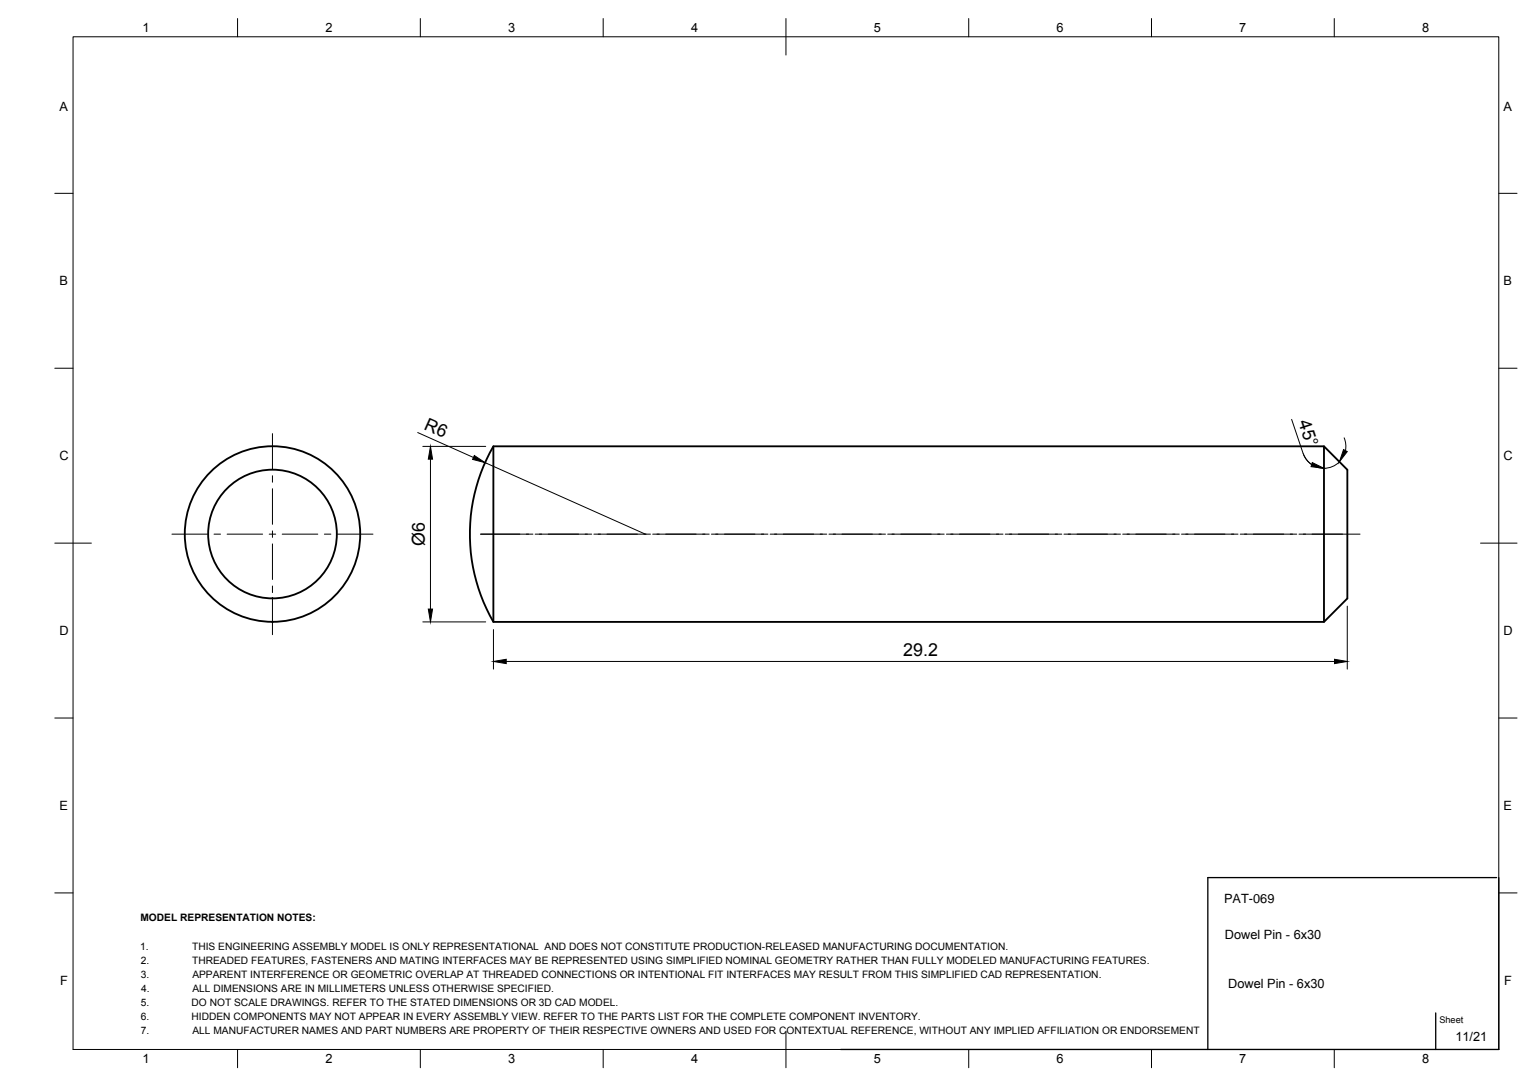
ISO-10303-21;
HEADER;
/* Generated by software containing ST-Developer
 * from STEP Tools, Inc. (www.steptools.com) 
 */

FILE_DESCRIPTION(
/* description */ ('Located fixture plate with toggle clamp'),
/* implementation_level */ '2;1');

FILE_NAME(
/* name */ 'Dowel Pin - 6x30.step',
/* time_stamp */ '2026-10-27T21:36:12-07:00',
/* author */ (''),
/* organization */ (''),
/* preprocessor_version */ 'ST-DEVELOPER v20.2',
/* originating_system */ 'Autodesk Translation Framework v15.17.0.0',
/* authorisation */ '');

FILE_SCHEMA (('AUTOMOTIVE_DESIGN { 1 0 10303 214 3 1 1 }'));
ENDSEC;

DATA;
#10=MECHANICAL_DESIGN_GEOMETRIC_PRESENTATION_REPRESENTATION('',(#330),#9285);
#202=SPHERICAL_SURFACE('',#5729,0.600000000000005);
#258=CONICAL_SURFACE('',#5733,0.26,0.785398163397448);
#282=SHAPE_REPRESENTATION_RELATIONSHIP('SRR','None',#9405,#306);
#306=ADVANCED_BREP_SHAPE_REPRESENTATION('',(#353),#9267);
#330=STYLED_ITEM('',(#9612),#353);
#353=MANIFOLD_SOLID_BREP('Body1',#5179);
#577=PLANE('',#5735);
#821=FACE_OUTER_BOUND('',#1202,.T.);
#822=FACE_OUTER_BOUND('',#1203,.T.);
#823=FACE_OUTER_BOUND('',#1204,.T.);
#824=FACE_OUTER_BOUND('',#1205,.T.);
#1202=EDGE_LOOP('',(#4188));
#1203=EDGE_LOOP('',(#4189,#4190,#4191,#4192));
#1204=EDGE_LOOP('',(#4193,#4194,#4195,#4196));
#1205=EDGE_LOOP('',(#4197));
#1491=CIRCLE('',#5730,0.3);
#1492=CIRCLE('',#5732,0.3);
#1493=CIRCLE('',#5734,0.22);
#1807=LINE('',#8361,#2217);
#1808=LINE('',#8365,#2218);
#2217=VECTOR('',#6799,0.3);
#2218=VECTOR('',#6804,0.26);
#2633=VERTEX_POINT('',#8356);
#2634=VERTEX_POINT('',#8359);
#2635=VERTEX_POINT('',#8363);
#3182=EDGE_CURVE('',#2633,#2633,#1491,.T.);
#3183=EDGE_CURVE('',#2634,#2634,#1492,.T.);
#3184=EDGE_CURVE('',#2634,#2633,#1807,.T.);
#3185=EDGE_CURVE('',#2635,#2635,#1493,.T.);
#3186=EDGE_CURVE('',#2635,#2634,#1808,.T.);
#4188=ORIENTED_EDGE('',*,*,#3182,.F.);
#4189=ORIENTED_EDGE('',*,*,#3183,.F.);
#4190=ORIENTED_EDGE('',*,*,#3184,.T.);
#4191=ORIENTED_EDGE('',*,*,#3182,.T.);
#4192=ORIENTED_EDGE('',*,*,#3184,.F.);
#4193=ORIENTED_EDGE('',*,*,#3185,.F.);
#4194=ORIENTED_EDGE('',*,*,#3186,.T.);
#4195=ORIENTED_EDGE('',*,*,#3183,.T.);
#4196=ORIENTED_EDGE('',*,*,#3186,.F.);
#4197=ORIENTED_EDGE('',*,*,#3185,.T.);
#4841=CYLINDRICAL_SURFACE('',#5731,0.3);
#5022=ADVANCED_FACE('',(#821),#202,.T.);
#5023=ADVANCED_FACE('',(#822),#4841,.T.);
#5024=ADVANCED_FACE('',(#823),#258,.T.);
#5025=ADVANCED_FACE('',(#824),#577,.T.);
#5179=CLOSED_SHELL('',(#5022,#5023,#5024,#5025));
#5728=AXIS2_PLACEMENT_3D('',#8354,#6789,#6790);
#5729=AXIS2_PLACEMENT_3D('',#8355,#6791,#6792);
#5730=AXIS2_PLACEMENT_3D('',#8357,#6793,#6794);
#5731=AXIS2_PLACEMENT_3D('',#8358,#6795,#6796);
#5732=AXIS2_PLACEMENT_3D('',#8360,#6797,#6798);
#5733=AXIS2_PLACEMENT_3D('',#8362,#6800,#6801);
#5734=AXIS2_PLACEMENT_3D('',#8364,#6802,#6803);
#5735=AXIS2_PLACEMENT_3D('',#8366,#6805,#6806);
#6789=DIRECTION('axis',(0.,0.,1.));
#6790=DIRECTION('refdir',(1.,0.,0.));
#6791=DIRECTION('center_axis',(6.12323399573677E-17,0.,1.));
#6792=DIRECTION('ref_axis',(1.,0.,0.));
#6793=DIRECTION('center_axis',(0.,-1.,0.));
#6794=DIRECTION('ref_axis',(1.,0.,0.));
#6795=DIRECTION('center_axis',(0.,-1.,0.));
#6796=DIRECTION('ref_axis',(1.,0.,0.));
#6797=DIRECTION('center_axis',(0.,-1.,0.));
#6798=DIRECTION('ref_axis',(1.,0.,0.));
#6799=DIRECTION('',(0.,1.,0.));
#6800=DIRECTION('center_axis',(0.,1.,0.));
#6801=DIRECTION('ref_axis',(1.,0.,0.));
#6802=DIRECTION('center_axis',(0.,-1.,0.));
#6803=DIRECTION('ref_axis',(1.,0.,0.));
#6804=DIRECTION('',(-0.707106781186547,0.707106781186548,-8.65956056235493E-17));
#6805=DIRECTION('center_axis',(0.,-1.,0.));
#6806=DIRECTION('ref_axis',(0.,0.,-1.));
#8354=CARTESIAN_POINT('',(0.,0.,0.));
#8355=CARTESIAN_POINT('Origin',(-8.04911692853238E-16,2.4,0.));
#8356=CARTESIAN_POINT('',(-0.3,2.91961524227066,-3.67394039744206E-17));
#8357=CARTESIAN_POINT('Origin',(0.,2.91961524227066,0.));
#8358=CARTESIAN_POINT('Origin',(0.,1.49980762113533,0.));
#8359=CARTESIAN_POINT('',(-0.3,0.0800000000000001,-3.67394039744206E-17));
#8360=CARTESIAN_POINT('Origin',(0.,0.08,0.));
#8361=CARTESIAN_POINT('',(-0.3,1.49980762113533,-3.67394039744206E-17));
#8362=CARTESIAN_POINT('Origin',(0.,0.04,0.));
#8363=CARTESIAN_POINT('',(-0.22,-6.93889390390723E-18,-2.69422295812418E-17));
#8364=CARTESIAN_POINT('Origin',(0.,0.,0.));
#8365=CARTESIAN_POINT('',(-0.26,0.04,-3.18408167778312E-17));
#8366=CARTESIAN_POINT('Origin',(0.,0.,0.));
#9237=UNCERTAINTY_MEASURE_WITH_UNIT(LENGTH_MEASURE(0.001),#9286,
'DISTANCE_ACCURACY_VALUE',
'Maximum model space distance between geometric entities at asserted c
onnectivities');
#9255=UNCERTAINTY_MEASURE_WITH_UNIT(LENGTH_MEASURE(0.001),#9286,
'DISTANCE_ACCURACY_VALUE',
'Maximum model space distance between geometric entities at asserted c
onnectivities');
#9267=(
GEOMETRIC_REPRESENTATION_CONTEXT(3)
GLOBAL_UNCERTAINTY_ASSIGNED_CONTEXT((#9237))
GLOBAL_UNIT_ASSIGNED_CONTEXT((#9286,#9288,#9289))
REPRESENTATION_CONTEXT('','3D')
);
#9285=(
GEOMETRIC_REPRESENTATION_CONTEXT(3)
GLOBAL_UNCERTAINTY_ASSIGNED_CONTEXT((#9255))
GLOBAL_UNIT_ASSIGNED_CONTEXT((#9286,#9288,#9289))
REPRESENTATION_CONTEXT('','3D')
);
#9286=(
LENGTH_UNIT()
NAMED_UNIT(*)
SI_UNIT(.CENTI.,.METRE.)
);
#9288=(
NAMED_UNIT(*)
PLANE_ANGLE_UNIT()
SI_UNIT($,.RADIAN.)
);
#9289=(
NAMED_UNIT(*)
SI_UNIT($,.STERADIAN.)
SOLID_ANGLE_UNIT()
);
#9301=SHAPE_DEFINITION_REPRESENTATION(#9330,#9405);
#9330=PRODUCT_DEFINITION_SHAPE('',$,#9435);
#9405=SHAPE_REPRESENTATION('',(#5728),#9267);
#9423=PRODUCT_DEFINITION_CONTEXT('part definition',#9512,'design');
#9435=PRODUCT_DEFINITION('Dowel Pin - 6x30','Dowel Pin - 6x30',#9464,#9423);
#9464=PRODUCT_DEFINITION_FORMATION('',$,#9525);
#9512=APPLICATION_CONTEXT(
'Core Data for Automotive Mechanical Design Process');
#9513=PRODUCT_CONTEXT('part definition',#9512,'mechanical');
#9525=PRODUCT('Dowel Pin - 6x30','Dowel Pin - 6x30','Dowel Pin - 6x30',
(#9513));
#9606=COLOUR_RGB('Grey',0.48,0.52,0.57);
#9607=FILL_AREA_STYLE_COLOUR('',#9606);
#9608=FILL_AREA_STYLE('',(#9607));
#9609=SURFACE_STYLE_FILL_AREA(#9608);
#9610=SURFACE_SIDE_STYLE('',(#9609));
#9611=SURFACE_STYLE_USAGE(.BOTH.,#9610);
#9612=PRESENTATION_STYLE_ASSIGNMENT((#9611));
ENDSEC;
END-ISO-10303-21;
